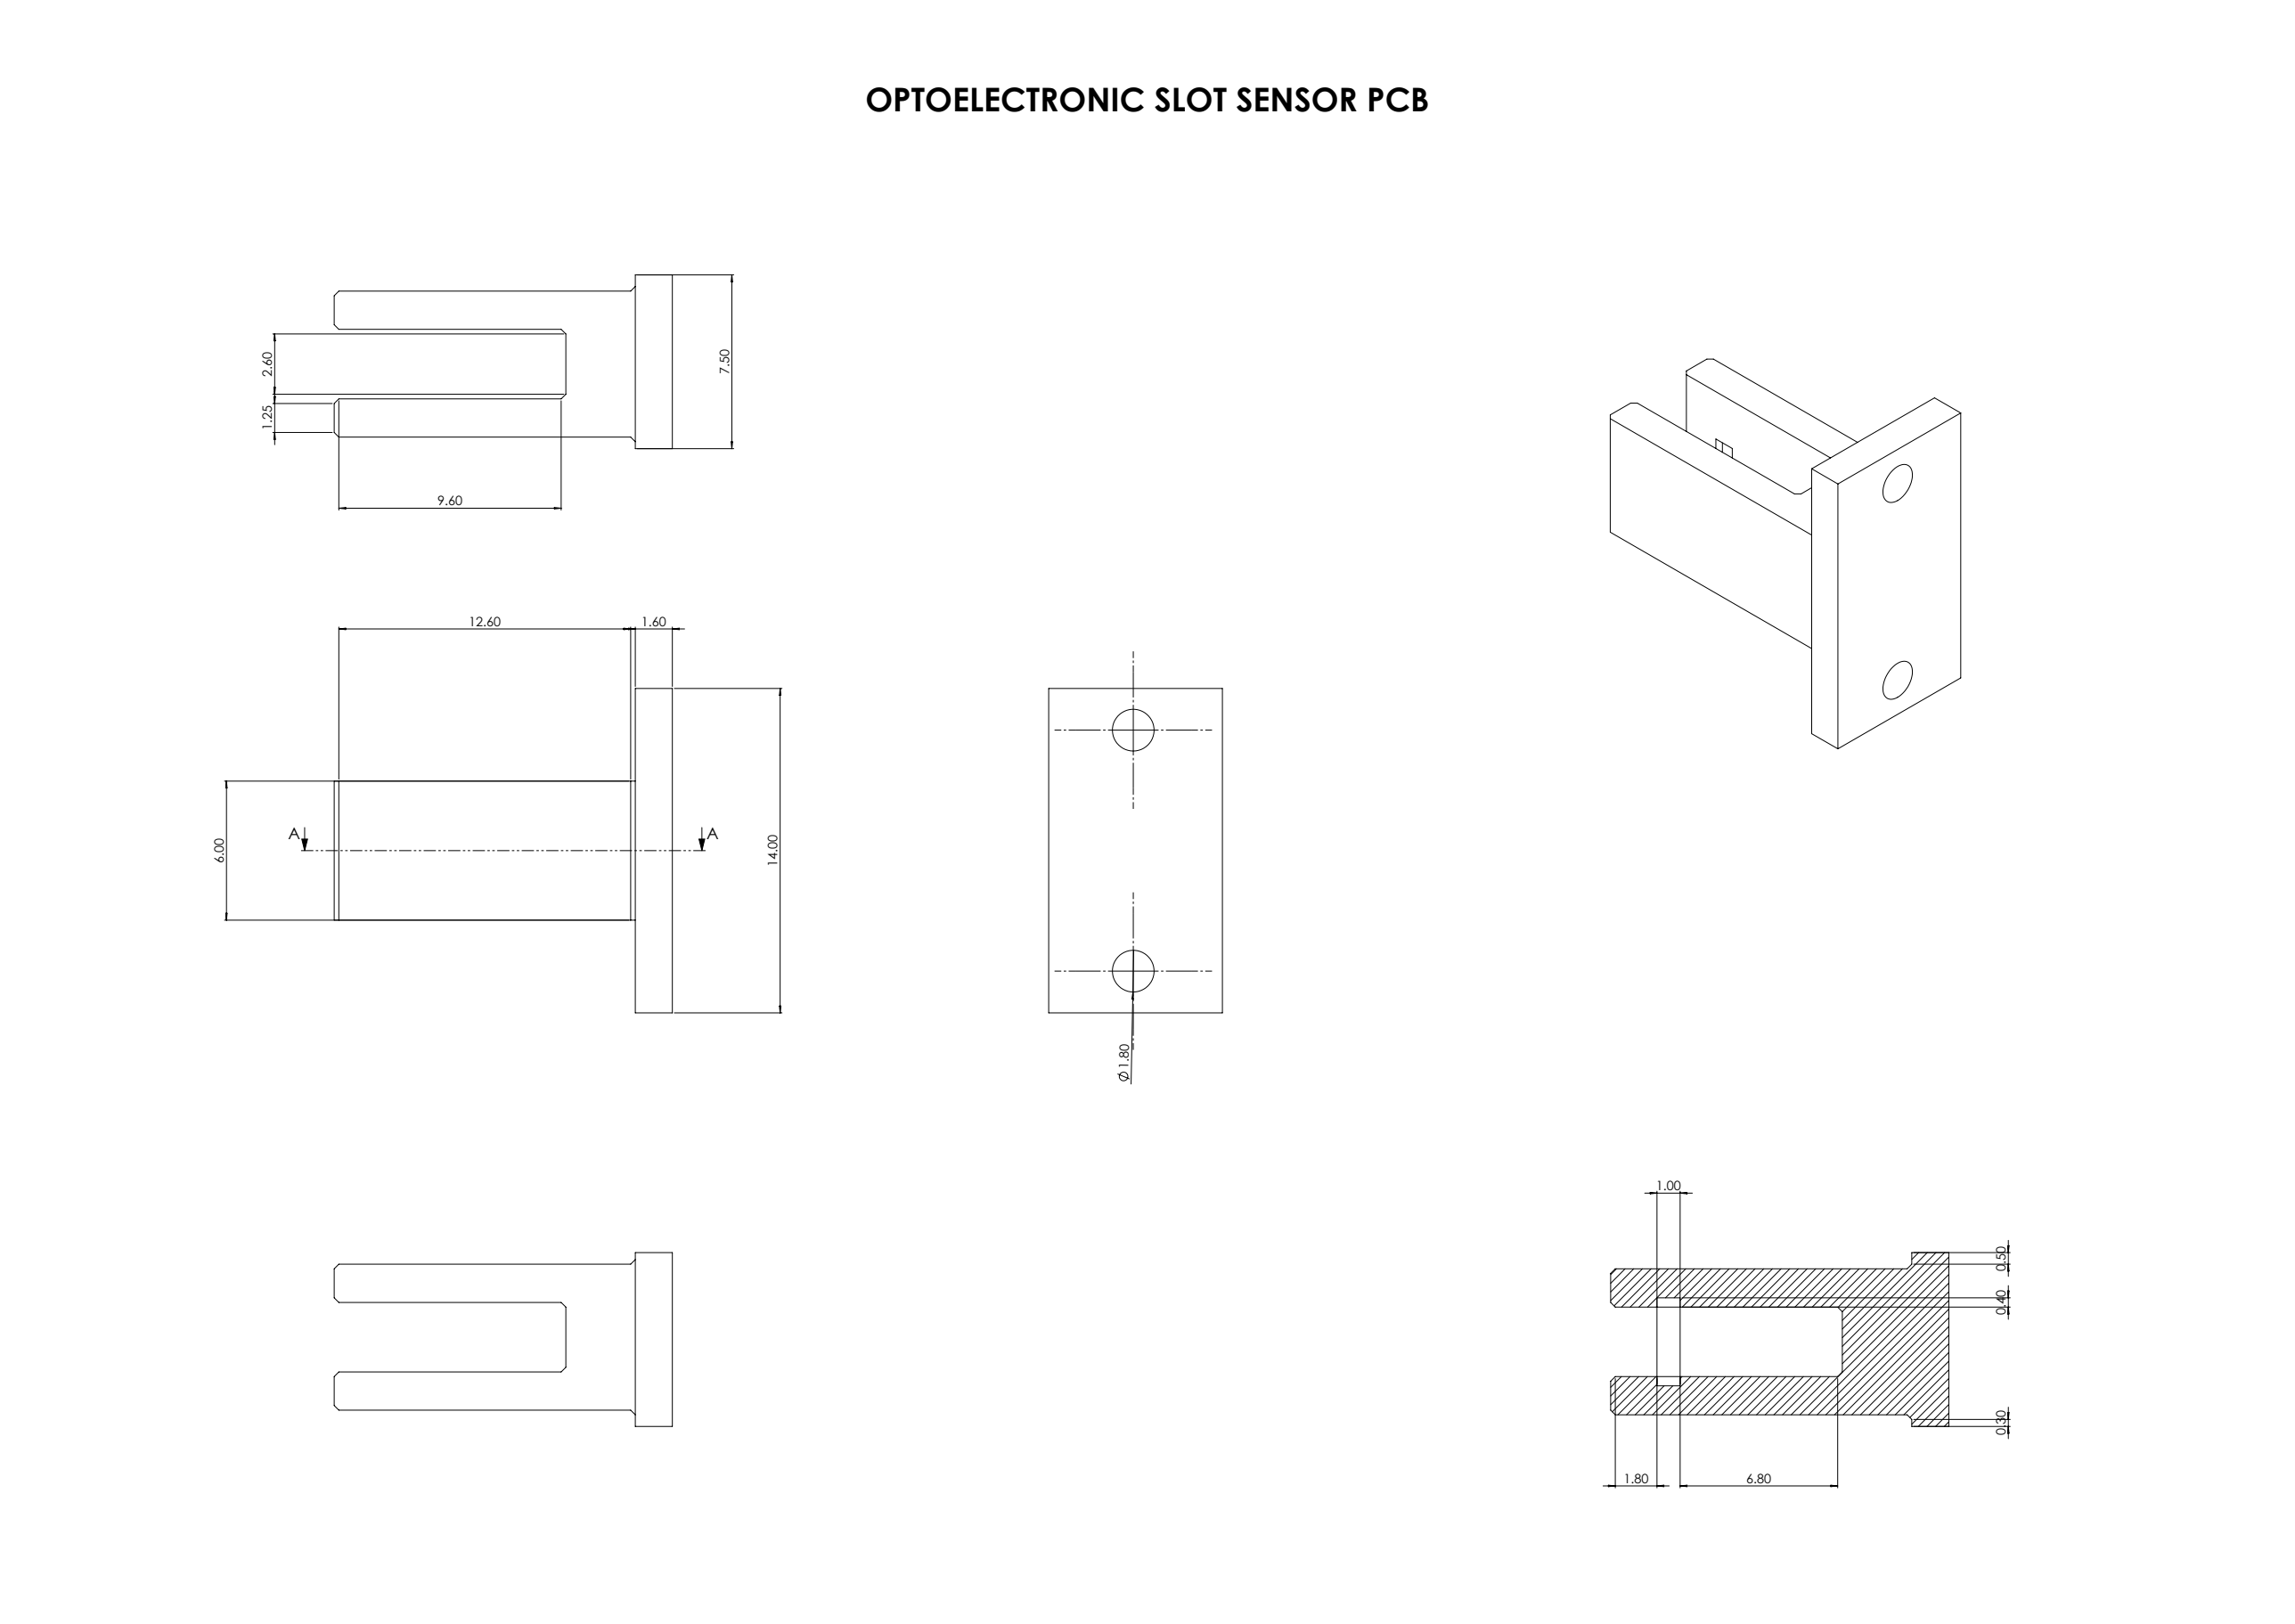
ISO-10303-21;
HEADER;
/* Generated by software containing ST-Developer
 * from STEP Tools, Inc. (www.steptools.com) 
 */

FILE_DESCRIPTION(
/* description */ (''),
/* implementation_level */ '2;1');

FILE_NAME(
/* name */ '11_Optoelectronic_Slot_Sensor_PCB.step',
/* time_stamp */ '2026-10-19T23:00:43-07:00',
/* author */ (''),
/* organization */ (''),
/* preprocessor_version */ 'ST-DEVELOPER v20.2',
/* originating_system */ 'Autodesk Translation Framework v15.15.0.0',
/* authorisation */ '');

FILE_SCHEMA (('AUTOMOTIVE_DESIGN { 1 0 10303 214 3 1 1 }'));
ENDSEC;

DATA;
#10=MECHANICAL_DESIGN_GEOMETRIC_PRESENTATION_REPRESENTATION('',(#1006),#55002);
#966=SHAPE_REPRESENTATION_RELATIONSHIP('SRR','None',#55114,#986);
#986=ADVANCED_BREP_SHAPE_REPRESENTATION('',(#1026),#54992);
#1006=STYLED_ITEM('',(#55379),#1026);
#1026=MANIFOLD_SOLID_BREP('Slot Sensor PCB',#24539);
#1232=FACE_BOUND('',#4568,.T.);
#1233=FACE_BOUND('',#4573,.T.);
#1234=FACE_BOUND('',#4577,.T.);
#1235=FACE_BOUND('',#4578,.T.);
#1236=FACE_BOUND('',#4579,.T.);
#1237=FACE_BOUND('',#4586,.T.);
#1238=FACE_BOUND('',#4587,.T.);
#1458=PLANE('',#26023);
#1459=PLANE('',#26024);
#1460=PLANE('',#26025);
#1461=PLANE('',#26026);
#1462=PLANE('',#26027);
#1463=PLANE('',#26028);
#1464=PLANE('',#26029);
#1465=PLANE('',#26030);
#1466=PLANE('',#26031);
#1467=PLANE('',#26032);
#1468=PLANE('',#26033);
#1469=PLANE('',#26034);
#1470=PLANE('',#26035);
#1471=PLANE('',#26036);
#1472=PLANE('',#26037);
#1473=PLANE('',#26040);
#1474=PLANE('',#26041);
#1475=PLANE('',#26046);
#1476=PLANE('',#26047);
#1477=PLANE('',#26048);
#1478=PLANE('',#26049);
#1479=PLANE('',#26050);
#1480=PLANE('',#26051);
#1481=PLANE('',#26052);
#1482=PLANE('',#26053);
#1483=PLANE('',#26054);
#1484=PLANE('',#26055);
#1485=PLANE('',#26056);
#1486=PLANE('',#26057);
#1487=PLANE('',#26058);
#1488=PLANE('',#26059);
#1489=PLANE('',#26060);
#1490=PLANE('',#26061);
#2178=CYLINDRICAL_SURFACE('',#26042,0.0900000000000001);
#2179=CYLINDRICAL_SURFACE('',#26044,0.09);
#3000=FACE_OUTER_BOUND('',#4560,.T.);
#3001=FACE_OUTER_BOUND('',#4561,.T.);
#3002=FACE_OUTER_BOUND('',#4562,.T.);
#3003=FACE_OUTER_BOUND('',#4563,.T.);
#3004=FACE_OUTER_BOUND('',#4564,.T.);
#3005=FACE_OUTER_BOUND('',#4565,.T.);
#3006=FACE_OUTER_BOUND('',#4566,.T.);
#3007=FACE_OUTER_BOUND('',#4567,.T.);
#3008=FACE_OUTER_BOUND('',#4569,.T.);
#3009=FACE_OUTER_BOUND('',#4570,.T.);
#3010=FACE_OUTER_BOUND('',#4571,.T.);
#3011=FACE_OUTER_BOUND('',#4572,.T.);
#3012=FACE_OUTER_BOUND('',#4574,.T.);
#3013=FACE_OUTER_BOUND('',#4575,.T.);
#3014=FACE_OUTER_BOUND('',#4576,.T.);
#3015=FACE_OUTER_BOUND('',#4580,.T.);
#3016=FACE_OUTER_BOUND('',#4581,.T.);
#3017=FACE_OUTER_BOUND('',#4582,.T.);
#3018=FACE_OUTER_BOUND('',#4583,.T.);
#3019=FACE_OUTER_BOUND('',#4584,.T.);
#3020=FACE_OUTER_BOUND('',#4585,.T.);
#3021=FACE_OUTER_BOUND('',#4588,.T.);
#3022=FACE_OUTER_BOUND('',#4589,.T.);
#3023=FACE_OUTER_BOUND('',#4590,.T.);
#3024=FACE_OUTER_BOUND('',#4591,.T.);
#3025=FACE_OUTER_BOUND('',#4592,.T.);
#3026=FACE_OUTER_BOUND('',#4593,.T.);
#3027=FACE_OUTER_BOUND('',#4594,.T.);
#3028=FACE_OUTER_BOUND('',#4595,.T.);
#3029=FACE_OUTER_BOUND('',#4596,.T.);
#3030=FACE_OUTER_BOUND('',#4597,.T.);
#3031=FACE_OUTER_BOUND('',#4598,.T.);
#3032=FACE_OUTER_BOUND('',#4599,.T.);
#3033=FACE_OUTER_BOUND('',#4600,.T.);
#3034=FACE_OUTER_BOUND('',#4601,.T.);
#4560=EDGE_LOOP('',(#18604,#18605,#18606,#18607));
#4561=EDGE_LOOP('',(#18608,#18609,#18610,#18611));
#4562=EDGE_LOOP('',(#18612,#18613,#18614,#18615,#18616,#18617,#18618,#18619,
#18620,#18621,#18622,#18623,#18624,#18625,#18626,#18627));
#4563=EDGE_LOOP('',(#18628,#18629,#18630,#18631));
#4564=EDGE_LOOP('',(#18632,#18633,#18634,#18635));
#4565=EDGE_LOOP('',(#18636,#18637,#18638,#18639,#18640,#18641,#18642,#18643,
#18644,#18645,#18646,#18647,#18648,#18649,#18650,#18651));
#4566=EDGE_LOOP('',(#18652,#18653,#18654,#18655));
#4567=EDGE_LOOP('',(#18656,#18657,#18658,#18659));
#4568=EDGE_LOOP('',(#18660,#18661,#18662,#18663));
#4569=EDGE_LOOP('',(#18664,#18665,#18666,#18667));
#4570=EDGE_LOOP('',(#18668,#18669,#18670,#18671));
#4571=EDGE_LOOP('',(#18672,#18673,#18674,#18675));
#4572=EDGE_LOOP('',(#18676,#18677,#18678,#18679));
#4573=EDGE_LOOP('',(#18680,#18681,#18682,#18683));
#4574=EDGE_LOOP('',(#18684,#18685,#18686,#18687));
#4575=EDGE_LOOP('',(#18688,#18689,#18690,#18691));
#4576=EDGE_LOOP('',(#18692,#18693,#18694,#18695));
#4577=EDGE_LOOP('',(#18696));
#4578=EDGE_LOOP('',(#18697));
#4579=EDGE_LOOP('',(#18698,#18699,#18700,#18701));
#4580=EDGE_LOOP('',(#18702,#18703,#18704,#18705));
#4581=EDGE_LOOP('',(#18706,#18707,#18708,#18709));
#4582=EDGE_LOOP('',(#18710,#18711,#18712,#18713));
#4583=EDGE_LOOP('',(#18714,#18715,#18716,#18717));
#4584=EDGE_LOOP('',(#18718,#18719,#18720,#18721));
#4585=EDGE_LOOP('',(#18722,#18723,#18724,#18725));
#4586=EDGE_LOOP('',(#18726));
#4587=EDGE_LOOP('',(#18727));
#4588=EDGE_LOOP('',(#18728,#18729,#18730,#18731));
#4589=EDGE_LOOP('',(#18732,#18733,#18734,#18735));
#4590=EDGE_LOOP('',(#18736,#18737,#18738,#18739));
#4591=EDGE_LOOP('',(#18740,#18741,#18742,#18743));
#4592=EDGE_LOOP('',(#18744,#18745,#18746,#18747));
#4593=EDGE_LOOP('',(#18748,#18749,#18750,#18751));
#4594=EDGE_LOOP('',(#18752,#18753,#18754,#18755));
#4595=EDGE_LOOP('',(#18756,#18757,#18758,#18759));
#4596=EDGE_LOOP('',(#18760,#18761,#18762,#18763));
#4597=EDGE_LOOP('',(#18764,#18765,#18766,#18767));
#4598=EDGE_LOOP('',(#18768,#18769,#18770,#18771));
#4599=EDGE_LOOP('',(#18772,#18773,#18774,#18775));
#4600=EDGE_LOOP('',(#18776,#18777,#18778,#18779));
#4601=EDGE_LOOP('',(#18780,#18781,#18782,#18783));
#6062=LINE('',#37264,#7883);
#6063=LINE('',#37266,#7884);
#6064=LINE('',#37268,#7885);
#6065=LINE('',#37269,#7886);
#6066=LINE('',#37272,#7887);
#6067=LINE('',#37274,#7888);
#6068=LINE('',#37275,#7889);
#6069=LINE('',#37278,#7890);
#6070=LINE('',#37280,#7891);
#6071=LINE('',#37282,#7892);
#6072=LINE('',#37284,#7893);
#6073=LINE('',#37286,#7894);
#6074=LINE('',#37288,#7895);
#6075=LINE('',#37290,#7896);
#6076=LINE('',#37292,#7897);
#6077=LINE('',#37294,#7898);
#6078=LINE('',#37296,#7899);
#6079=LINE('',#37298,#7900);
#6080=LINE('',#37300,#7901);
#6081=LINE('',#37302,#7902);
#6082=LINE('',#37303,#7903);
#6083=LINE('',#37306,#7904);
#6084=LINE('',#37308,#7905);
#6085=LINE('',#37309,#7906);
#6086=LINE('',#37312,#7907);
#6087=LINE('',#37313,#7908);
#6088=LINE('',#37316,#7909);
#6089=LINE('',#37318,#7910);
#6090=LINE('',#37320,#7911);
#6091=LINE('',#37322,#7912);
#6092=LINE('',#37324,#7913);
#6093=LINE('',#37326,#7914);
#6094=LINE('',#37327,#7915);
#6095=LINE('',#37329,#7916);
#6096=LINE('',#37331,#7917);
#6097=LINE('',#37333,#7918);
#6098=LINE('',#37335,#7919);
#6099=LINE('',#37336,#7920);
#6100=LINE('',#37338,#7921);
#6101=LINE('',#37340,#7922);
#6102=LINE('',#37343,#7923);
#6103=LINE('',#37345,#7924);
#6104=LINE('',#37347,#7925);
#6105=LINE('',#37348,#7926);
#6106=LINE('',#37350,#7927);
#6107=LINE('',#37352,#7928);
#6108=LINE('',#37354,#7929);
#6109=LINE('',#37356,#7930);
#6110=LINE('',#37359,#7931);
#6111=LINE('',#37361,#7932);
#6112=LINE('',#37363,#7933);
#6113=LINE('',#37364,#7934);
#6114=LINE('',#37367,#7935);
#6115=LINE('',#37368,#7936);
#6116=LINE('',#37372,#7937);
#6117=LINE('',#37374,#7938);
#6118=LINE('',#37376,#7939);
#6119=LINE('',#37377,#7940);
#6120=LINE('',#37382,#7941);
#6121=LINE('',#37384,#7942);
#6122=LINE('',#37389,#7943);
#6123=LINE('',#37393,#7944);
#6124=LINE('',#37396,#7945);
#6125=LINE('',#37398,#7946);
#6126=LINE('',#37399,#7947);
#6127=LINE('',#37402,#7948);
#6128=LINE('',#37404,#7949);
#6129=LINE('',#37405,#7950);
#6130=LINE('',#37407,#7951);
#6131=LINE('',#37408,#7952);
#6132=LINE('',#37414,#7953);
#6133=LINE('',#37415,#7954);
#6134=LINE('',#37416,#7955);
#6135=LINE('',#37419,#7956);
#6136=LINE('',#37420,#7957);
#6137=LINE('',#37423,#7958);
#6138=LINE('',#37424,#7959);
#6139=LINE('',#37426,#7960);
#6140=LINE('',#37430,#7961);
#6141=LINE('',#37432,#7962);
#6142=LINE('',#37433,#7963);
#6143=LINE('',#37436,#7964);
#6144=LINE('',#37437,#7965);
#6145=LINE('',#37440,#7966);
#6146=LINE('',#37441,#7967);
#6147=LINE('',#37443,#7968);
#7883=VECTOR('',#30386,1.);
#7884=VECTOR('',#30387,1.);
#7885=VECTOR('',#30388,1.);
#7886=VECTOR('',#30389,1.);
#7887=VECTOR('',#30392,1.);
#7888=VECTOR('',#30393,1.);
#7889=VECTOR('',#30394,1.);
#7890=VECTOR('',#30397,1.);
#7891=VECTOR('',#30398,1.);
#7892=VECTOR('',#30399,1.);
#7893=VECTOR('',#30400,1.);
#7894=VECTOR('',#30401,1.);
#7895=VECTOR('',#30402,1.);
#7896=VECTOR('',#30403,1.);
#7897=VECTOR('',#30404,1.);
#7898=VECTOR('',#30405,1.);
#7899=VECTOR('',#30406,1.);
#7900=VECTOR('',#30407,1.);
#7901=VECTOR('',#30408,1.);
#7902=VECTOR('',#30409,1.);
#7903=VECTOR('',#30410,1.);
#7904=VECTOR('',#30413,1.);
#7905=VECTOR('',#30414,1.);
#7906=VECTOR('',#30415,1.);
#7907=VECTOR('',#30418,1.);
#7908=VECTOR('',#30419,1.);
#7909=VECTOR('',#30422,1.);
#7910=VECTOR('',#30423,1.);
#7911=VECTOR('',#30424,1.);
#7912=VECTOR('',#30425,1.);
#7913=VECTOR('',#30426,1.);
#7914=VECTOR('',#30427,1.);
#7915=VECTOR('',#30428,1.);
#7916=VECTOR('',#30429,1.);
#7917=VECTOR('',#30430,1.);
#7918=VECTOR('',#30431,1.);
#7919=VECTOR('',#30432,1.);
#7920=VECTOR('',#30433,1.);
#7921=VECTOR('',#30436,1.);
#7922=VECTOR('',#30439,1.);
#7923=VECTOR('',#30440,1.);
#7924=VECTOR('',#30441,1.);
#7925=VECTOR('',#30442,1.);
#7926=VECTOR('',#30443,1.);
#7927=VECTOR('',#30446,1.);
#7928=VECTOR('',#30449,1.);
#7929=VECTOR('',#30452,1.);
#7930=VECTOR('',#30455,1.);
#7931=VECTOR('',#30456,1.);
#7932=VECTOR('',#30457,1.);
#7933=VECTOR('',#30458,1.);
#7934=VECTOR('',#30459,1.);
#7935=VECTOR('',#30464,1.);
#7936=VECTOR('',#30465,1.);
#7937=VECTOR('',#30468,1.);
#7938=VECTOR('',#30469,1.);
#7939=VECTOR('',#30470,1.);
#7940=VECTOR('',#30471,1.);
#7941=VECTOR('',#30476,1.);
#7942=VECTOR('',#30479,1.);
#7943=VECTOR('',#30486,0.0900000000000001);
#7944=VECTOR('',#30491,0.09);
#7945=VECTOR('',#30494,1.);
#7946=VECTOR('',#30495,1.);
#7947=VECTOR('',#30496,1.);
#7948=VECTOR('',#30499,1.);
#7949=VECTOR('',#30500,1.);
#7950=VECTOR('',#30501,1.);
#7951=VECTOR('',#30504,1.);
#7952=VECTOR('',#30505,1.);
#7953=VECTOR('',#30512,1.);
#7954=VECTOR('',#30513,1.);
#7955=VECTOR('',#30514,1.);
#7956=VECTOR('',#30517,1.);
#7957=VECTOR('',#30518,1.);
#7958=VECTOR('',#30521,1.);
#7959=VECTOR('',#30522,1.);
#7960=VECTOR('',#30525,1.);
#7961=VECTOR('',#30530,1.);
#7962=VECTOR('',#30531,1.);
#7963=VECTOR('',#30532,1.);
#7964=VECTOR('',#30535,1.);
#7965=VECTOR('',#30536,1.);
#7966=VECTOR('',#30539,1.);
#7967=VECTOR('',#30540,1.);
#7968=VECTOR('',#30543,1.);
#9678=CIRCLE('',#26038,0.09);
#9679=CIRCLE('',#26039,0.0900000000000001);
#9680=CIRCLE('',#26043,0.0900000000000001);
#9681=CIRCLE('',#26045,0.09);
#10905=VERTEX_POINT('',#37262);
#10906=VERTEX_POINT('',#37263);
#10907=VERTEX_POINT('',#37265);
#10908=VERTEX_POINT('',#37267);
#10909=VERTEX_POINT('',#37271);
#10910=VERTEX_POINT('',#37273);
#10911=VERTEX_POINT('',#37277);
#10912=VERTEX_POINT('',#37279);
#10913=VERTEX_POINT('',#37281);
#10914=VERTEX_POINT('',#37283);
#10915=VERTEX_POINT('',#37285);
#10916=VERTEX_POINT('',#37287);
#10917=VERTEX_POINT('',#37289);
#10918=VERTEX_POINT('',#37291);
#10919=VERTEX_POINT('',#37293);
#10920=VERTEX_POINT('',#37295);
#10921=VERTEX_POINT('',#37297);
#10922=VERTEX_POINT('',#37299);
#10923=VERTEX_POINT('',#37301);
#10924=VERTEX_POINT('',#37305);
#10925=VERTEX_POINT('',#37307);
#10926=VERTEX_POINT('',#37311);
#10927=VERTEX_POINT('',#37315);
#10928=VERTEX_POINT('',#37317);
#10929=VERTEX_POINT('',#37319);
#10930=VERTEX_POINT('',#37321);
#10931=VERTEX_POINT('',#37323);
#10932=VERTEX_POINT('',#37325);
#10933=VERTEX_POINT('',#37328);
#10934=VERTEX_POINT('',#37330);
#10935=VERTEX_POINT('',#37332);
#10936=VERTEX_POINT('',#37334);
#10937=VERTEX_POINT('',#37341);
#10938=VERTEX_POINT('',#37342);
#10939=VERTEX_POINT('',#37344);
#10940=VERTEX_POINT('',#37346);
#10941=VERTEX_POINT('',#37357);
#10942=VERTEX_POINT('',#37358);
#10943=VERTEX_POINT('',#37360);
#10944=VERTEX_POINT('',#37362);
#10945=VERTEX_POINT('',#37370);
#10946=VERTEX_POINT('',#37371);
#10947=VERTEX_POINT('',#37373);
#10948=VERTEX_POINT('',#37375);
#10949=VERTEX_POINT('',#37378);
#10950=VERTEX_POINT('',#37380);
#10951=VERTEX_POINT('',#37387);
#10952=VERTEX_POINT('',#37391);
#10953=VERTEX_POINT('',#37395);
#10954=VERTEX_POINT('',#37397);
#10955=VERTEX_POINT('',#37401);
#10956=VERTEX_POINT('',#37403);
#10957=VERTEX_POINT('',#37412);
#10958=VERTEX_POINT('',#37413);
#10959=VERTEX_POINT('',#37418);
#10960=VERTEX_POINT('',#37422);
#10961=VERTEX_POINT('',#37429);
#10962=VERTEX_POINT('',#37431);
#10963=VERTEX_POINT('',#37435);
#10964=VERTEX_POINT('',#37439);
#13710=EDGE_CURVE('',#10905,#10906,#6062,.T.);
#13711=EDGE_CURVE('',#10906,#10907,#6063,.T.);
#13712=EDGE_CURVE('',#10907,#10908,#6064,.T.);
#13713=EDGE_CURVE('',#10908,#10905,#6065,.T.);
#13714=EDGE_CURVE('',#10906,#10909,#6066,.T.);
#13715=EDGE_CURVE('',#10910,#10909,#6067,.T.);
#13716=EDGE_CURVE('',#10907,#10910,#6068,.T.);
#13717=EDGE_CURVE('',#10905,#10911,#6069,.T.);
#13718=EDGE_CURVE('',#10912,#10911,#6070,.T.);
#13719=EDGE_CURVE('',#10912,#10913,#6071,.T.);
#13720=EDGE_CURVE('',#10914,#10913,#6072,.T.);
#13721=EDGE_CURVE('',#10915,#10914,#6073,.T.);
#13722=EDGE_CURVE('',#10916,#10915,#6074,.T.);
#13723=EDGE_CURVE('',#10917,#10916,#6075,.T.);
#13724=EDGE_CURVE('',#10918,#10917,#6076,.T.);
#13725=EDGE_CURVE('',#10918,#10919,#6077,.T.);
#13726=EDGE_CURVE('',#10920,#10919,#6078,.T.);
#13727=EDGE_CURVE('',#10920,#10921,#6079,.T.);
#13728=EDGE_CURVE('',#10922,#10921,#6080,.T.);
#13729=EDGE_CURVE('',#10922,#10923,#6081,.T.);
#13730=EDGE_CURVE('',#10909,#10923,#6082,.T.);
#13731=EDGE_CURVE('',#10915,#10924,#6083,.T.);
#13732=EDGE_CURVE('',#10924,#10925,#6084,.T.);
#13733=EDGE_CURVE('',#10925,#10916,#6085,.T.);
#13734=EDGE_CURVE('',#10926,#10925,#6086,.T.);
#13735=EDGE_CURVE('',#10917,#10926,#6087,.T.);
#13736=EDGE_CURVE('',#10927,#10910,#6088,.T.);
#13737=EDGE_CURVE('',#10927,#10928,#6089,.T.);
#13738=EDGE_CURVE('',#10929,#10928,#6090,.T.);
#13739=EDGE_CURVE('',#10929,#10930,#6091,.T.);
#13740=EDGE_CURVE('',#10931,#10930,#6092,.T.);
#13741=EDGE_CURVE('',#10931,#10932,#6093,.T.);
#13742=EDGE_CURVE('',#10926,#10932,#6094,.T.);
#13743=EDGE_CURVE('',#10933,#10924,#6095,.T.);
#13744=EDGE_CURVE('',#10934,#10933,#6096,.T.);
#13745=EDGE_CURVE('',#10935,#10934,#6097,.T.);
#13746=EDGE_CURVE('',#10936,#10935,#6098,.T.);
#13747=EDGE_CURVE('',#10936,#10908,#6099,.T.);
#13748=EDGE_CURVE('',#10923,#10927,#6100,.T.);
#13749=EDGE_CURVE('',#10928,#10922,#6101,.T.);
#13750=EDGE_CURVE('',#10937,#10938,#6102,.T.);
#13751=EDGE_CURVE('',#10938,#10939,#6103,.T.);
#13752=EDGE_CURVE('',#10939,#10940,#6104,.T.);
#13753=EDGE_CURVE('',#10940,#10937,#6105,.T.);
#13754=EDGE_CURVE('',#10921,#10929,#6106,.T.);
#13755=EDGE_CURVE('',#10930,#10920,#6107,.T.);
#13756=EDGE_CURVE('',#10932,#10918,#6108,.T.);
#13757=EDGE_CURVE('',#10919,#10931,#6109,.T.);
#13758=EDGE_CURVE('',#10941,#10942,#6110,.T.);
#13759=EDGE_CURVE('',#10942,#10943,#6111,.T.);
#13760=EDGE_CURVE('',#10943,#10944,#6112,.T.);
#13761=EDGE_CURVE('',#10944,#10941,#6113,.T.);
#13762=EDGE_CURVE('',#10913,#10934,#6114,.T.);
#13763=EDGE_CURVE('',#10933,#10914,#6115,.T.);
#13764=EDGE_CURVE('',#10945,#10946,#6116,.T.);
#13765=EDGE_CURVE('',#10946,#10947,#6117,.T.);
#13766=EDGE_CURVE('',#10948,#10947,#6118,.T.);
#13767=EDGE_CURVE('',#10945,#10948,#6119,.T.);
#13768=EDGE_CURVE('',#10949,#10949,#9678,.T.);
#13769=EDGE_CURVE('',#10950,#10950,#9679,.T.);
#13770=EDGE_CURVE('',#10935,#10912,#6120,.T.);
#13771=EDGE_CURVE('',#10911,#10936,#6121,.T.);
#13772=EDGE_CURVE('',#10951,#10951,#9680,.T.);
#13773=EDGE_CURVE('',#10951,#10950,#6122,.T.);
#13774=EDGE_CURVE('',#10952,#10952,#9681,.T.);
#13775=EDGE_CURVE('',#10952,#10949,#6123,.T.);
#13776=EDGE_CURVE('',#10953,#10945,#6124,.T.);
#13777=EDGE_CURVE('',#10954,#10948,#6125,.T.);
#13778=EDGE_CURVE('',#10953,#10954,#6126,.T.);
#13779=EDGE_CURVE('',#10955,#10953,#6127,.T.);
#13780=EDGE_CURVE('',#10956,#10954,#6128,.T.);
#13781=EDGE_CURVE('',#10955,#10956,#6129,.T.);
#13782=EDGE_CURVE('',#10946,#10955,#6130,.T.);
#13783=EDGE_CURVE('',#10947,#10956,#6131,.T.);
#13784=EDGE_CURVE('',#10957,#10958,#6132,.T.);
#13785=EDGE_CURVE('',#10957,#10938,#6133,.T.);
#13786=EDGE_CURVE('',#10958,#10937,#6134,.T.);
#13787=EDGE_CURVE('',#10959,#10957,#6135,.T.);
#13788=EDGE_CURVE('',#10959,#10939,#6136,.T.);
#13789=EDGE_CURVE('',#10960,#10959,#6137,.T.);
#13790=EDGE_CURVE('',#10960,#10940,#6138,.T.);
#13791=EDGE_CURVE('',#10958,#10960,#6139,.T.);
#13792=EDGE_CURVE('',#10941,#10961,#6140,.T.);
#13793=EDGE_CURVE('',#10961,#10962,#6141,.T.);
#13794=EDGE_CURVE('',#10942,#10962,#6142,.T.);
#13795=EDGE_CURVE('',#10944,#10963,#6143,.T.);
#13796=EDGE_CURVE('',#10963,#10961,#6144,.T.);
#13797=EDGE_CURVE('',#10943,#10964,#6145,.T.);
#13798=EDGE_CURVE('',#10964,#10963,#6146,.T.);
#13799=EDGE_CURVE('',#10962,#10964,#6147,.T.);
#18604=ORIENTED_EDGE('',*,*,#13710,.T.);
#18605=ORIENTED_EDGE('',*,*,#13711,.T.);
#18606=ORIENTED_EDGE('',*,*,#13712,.T.);
#18607=ORIENTED_EDGE('',*,*,#13713,.T.);
#18608=ORIENTED_EDGE('',*,*,#13711,.F.);
#18609=ORIENTED_EDGE('',*,*,#13714,.T.);
#18610=ORIENTED_EDGE('',*,*,#13715,.F.);
#18611=ORIENTED_EDGE('',*,*,#13716,.F.);
#18612=ORIENTED_EDGE('',*,*,#13710,.F.);
#18613=ORIENTED_EDGE('',*,*,#13717,.T.);
#18614=ORIENTED_EDGE('',*,*,#13718,.F.);
#18615=ORIENTED_EDGE('',*,*,#13719,.T.);
#18616=ORIENTED_EDGE('',*,*,#13720,.F.);
#18617=ORIENTED_EDGE('',*,*,#13721,.F.);
#18618=ORIENTED_EDGE('',*,*,#13722,.F.);
#18619=ORIENTED_EDGE('',*,*,#13723,.F.);
#18620=ORIENTED_EDGE('',*,*,#13724,.F.);
#18621=ORIENTED_EDGE('',*,*,#13725,.T.);
#18622=ORIENTED_EDGE('',*,*,#13726,.F.);
#18623=ORIENTED_EDGE('',*,*,#13727,.T.);
#18624=ORIENTED_EDGE('',*,*,#13728,.F.);
#18625=ORIENTED_EDGE('',*,*,#13729,.T.);
#18626=ORIENTED_EDGE('',*,*,#13730,.F.);
#18627=ORIENTED_EDGE('',*,*,#13714,.F.);
#18628=ORIENTED_EDGE('',*,*,#13722,.T.);
#18629=ORIENTED_EDGE('',*,*,#13731,.T.);
#18630=ORIENTED_EDGE('',*,*,#13732,.T.);
#18631=ORIENTED_EDGE('',*,*,#13733,.T.);
#18632=ORIENTED_EDGE('',*,*,#13733,.F.);
#18633=ORIENTED_EDGE('',*,*,#13734,.F.);
#18634=ORIENTED_EDGE('',*,*,#13735,.F.);
#18635=ORIENTED_EDGE('',*,*,#13723,.T.);
#18636=ORIENTED_EDGE('',*,*,#13712,.F.);
#18637=ORIENTED_EDGE('',*,*,#13716,.T.);
#18638=ORIENTED_EDGE('',*,*,#13736,.F.);
#18639=ORIENTED_EDGE('',*,*,#13737,.T.);
#18640=ORIENTED_EDGE('',*,*,#13738,.F.);
#18641=ORIENTED_EDGE('',*,*,#13739,.T.);
#18642=ORIENTED_EDGE('',*,*,#13740,.F.);
#18643=ORIENTED_EDGE('',*,*,#13741,.T.);
#18644=ORIENTED_EDGE('',*,*,#13742,.F.);
#18645=ORIENTED_EDGE('',*,*,#13734,.T.);
#18646=ORIENTED_EDGE('',*,*,#13732,.F.);
#18647=ORIENTED_EDGE('',*,*,#13743,.F.);
#18648=ORIENTED_EDGE('',*,*,#13744,.F.);
#18649=ORIENTED_EDGE('',*,*,#13745,.F.);
#18650=ORIENTED_EDGE('',*,*,#13746,.F.);
#18651=ORIENTED_EDGE('',*,*,#13747,.T.);
#18652=ORIENTED_EDGE('',*,*,#13736,.T.);
#18653=ORIENTED_EDGE('',*,*,#13715,.T.);
#18654=ORIENTED_EDGE('',*,*,#13730,.T.);
#18655=ORIENTED_EDGE('',*,*,#13748,.T.);
#18656=ORIENTED_EDGE('',*,*,#13748,.F.);
#18657=ORIENTED_EDGE('',*,*,#13729,.F.);
#18658=ORIENTED_EDGE('',*,*,#13749,.F.);
#18659=ORIENTED_EDGE('',*,*,#13737,.F.);
#18660=ORIENTED_EDGE('',*,*,#13750,.T.);
#18661=ORIENTED_EDGE('',*,*,#13751,.T.);
#18662=ORIENTED_EDGE('',*,*,#13752,.T.);
#18663=ORIENTED_EDGE('',*,*,#13753,.T.);
#18664=ORIENTED_EDGE('',*,*,#13728,.T.);
#18665=ORIENTED_EDGE('',*,*,#13754,.T.);
#18666=ORIENTED_EDGE('',*,*,#13738,.T.);
#18667=ORIENTED_EDGE('',*,*,#13749,.T.);
#18668=ORIENTED_EDGE('',*,*,#13754,.F.);
#18669=ORIENTED_EDGE('',*,*,#13727,.F.);
#18670=ORIENTED_EDGE('',*,*,#13755,.F.);
#18671=ORIENTED_EDGE('',*,*,#13739,.F.);
#18672=ORIENTED_EDGE('',*,*,#13724,.T.);
#18673=ORIENTED_EDGE('',*,*,#13735,.T.);
#18674=ORIENTED_EDGE('',*,*,#13742,.T.);
#18675=ORIENTED_EDGE('',*,*,#13756,.T.);
#18676=ORIENTED_EDGE('',*,*,#13756,.F.);
#18677=ORIENTED_EDGE('',*,*,#13741,.F.);
#18678=ORIENTED_EDGE('',*,*,#13757,.F.);
#18679=ORIENTED_EDGE('',*,*,#13725,.F.);
#18680=ORIENTED_EDGE('',*,*,#13758,.T.);
#18681=ORIENTED_EDGE('',*,*,#13759,.T.);
#18682=ORIENTED_EDGE('',*,*,#13760,.T.);
#18683=ORIENTED_EDGE('',*,*,#13761,.T.);
#18684=ORIENTED_EDGE('',*,*,#13726,.T.);
#18685=ORIENTED_EDGE('',*,*,#13757,.T.);
#18686=ORIENTED_EDGE('',*,*,#13740,.T.);
#18687=ORIENTED_EDGE('',*,*,#13755,.T.);
#18688=ORIENTED_EDGE('',*,*,#13720,.T.);
#18689=ORIENTED_EDGE('',*,*,#13762,.T.);
#18690=ORIENTED_EDGE('',*,*,#13744,.T.);
#18691=ORIENTED_EDGE('',*,*,#13763,.T.);
#18692=ORIENTED_EDGE('',*,*,#13764,.T.);
#18693=ORIENTED_EDGE('',*,*,#13765,.T.);
#18694=ORIENTED_EDGE('',*,*,#13766,.F.);
#18695=ORIENTED_EDGE('',*,*,#13767,.F.);
#18696=ORIENTED_EDGE('',*,*,#13768,.T.);
#18697=ORIENTED_EDGE('',*,*,#13769,.T.);
#18698=ORIENTED_EDGE('',*,*,#13745,.T.);
#18699=ORIENTED_EDGE('',*,*,#13762,.F.);
#18700=ORIENTED_EDGE('',*,*,#13719,.F.);
#18701=ORIENTED_EDGE('',*,*,#13770,.F.);
#18702=ORIENTED_EDGE('',*,*,#13718,.T.);
#18703=ORIENTED_EDGE('',*,*,#13771,.T.);
#18704=ORIENTED_EDGE('',*,*,#13746,.T.);
#18705=ORIENTED_EDGE('',*,*,#13770,.T.);
#18706=ORIENTED_EDGE('',*,*,#13713,.F.);
#18707=ORIENTED_EDGE('',*,*,#13747,.F.);
#18708=ORIENTED_EDGE('',*,*,#13771,.F.);
#18709=ORIENTED_EDGE('',*,*,#13717,.F.);
#18710=ORIENTED_EDGE('',*,*,#13772,.F.);
#18711=ORIENTED_EDGE('',*,*,#13773,.T.);
#18712=ORIENTED_EDGE('',*,*,#13769,.F.);
#18713=ORIENTED_EDGE('',*,*,#13773,.F.);
#18714=ORIENTED_EDGE('',*,*,#13774,.F.);
#18715=ORIENTED_EDGE('',*,*,#13775,.T.);
#18716=ORIENTED_EDGE('',*,*,#13768,.F.);
#18717=ORIENTED_EDGE('',*,*,#13775,.F.);
#18718=ORIENTED_EDGE('',*,*,#13776,.T.);
#18719=ORIENTED_EDGE('',*,*,#13767,.T.);
#18720=ORIENTED_EDGE('',*,*,#13777,.F.);
#18721=ORIENTED_EDGE('',*,*,#13778,.F.);
#18722=ORIENTED_EDGE('',*,*,#13779,.T.);
#18723=ORIENTED_EDGE('',*,*,#13778,.T.);
#18724=ORIENTED_EDGE('',*,*,#13780,.F.);
#18725=ORIENTED_EDGE('',*,*,#13781,.F.);
#18726=ORIENTED_EDGE('',*,*,#13772,.T.);
#18727=ORIENTED_EDGE('',*,*,#13774,.T.);
#18728=ORIENTED_EDGE('',*,*,#13782,.T.);
#18729=ORIENTED_EDGE('',*,*,#13781,.T.);
#18730=ORIENTED_EDGE('',*,*,#13783,.F.);
#18731=ORIENTED_EDGE('',*,*,#13765,.F.);
#18732=ORIENTED_EDGE('',*,*,#13766,.T.);
#18733=ORIENTED_EDGE('',*,*,#13783,.T.);
#18734=ORIENTED_EDGE('',*,*,#13780,.T.);
#18735=ORIENTED_EDGE('',*,*,#13777,.T.);
#18736=ORIENTED_EDGE('',*,*,#13764,.F.);
#18737=ORIENTED_EDGE('',*,*,#13776,.F.);
#18738=ORIENTED_EDGE('',*,*,#13779,.F.);
#18739=ORIENTED_EDGE('',*,*,#13782,.F.);
#18740=ORIENTED_EDGE('',*,*,#13784,.F.);
#18741=ORIENTED_EDGE('',*,*,#13785,.T.);
#18742=ORIENTED_EDGE('',*,*,#13750,.F.);
#18743=ORIENTED_EDGE('',*,*,#13786,.F.);
#18744=ORIENTED_EDGE('',*,*,#13787,.F.);
#18745=ORIENTED_EDGE('',*,*,#13788,.T.);
#18746=ORIENTED_EDGE('',*,*,#13751,.F.);
#18747=ORIENTED_EDGE('',*,*,#13785,.F.);
#18748=ORIENTED_EDGE('',*,*,#13789,.F.);
#18749=ORIENTED_EDGE('',*,*,#13790,.T.);
#18750=ORIENTED_EDGE('',*,*,#13752,.F.);
#18751=ORIENTED_EDGE('',*,*,#13788,.F.);
#18752=ORIENTED_EDGE('',*,*,#13791,.F.);
#18753=ORIENTED_EDGE('',*,*,#13786,.T.);
#18754=ORIENTED_EDGE('',*,*,#13753,.F.);
#18755=ORIENTED_EDGE('',*,*,#13790,.F.);
#18756=ORIENTED_EDGE('',*,*,#13791,.T.);
#18757=ORIENTED_EDGE('',*,*,#13789,.T.);
#18758=ORIENTED_EDGE('',*,*,#13787,.T.);
#18759=ORIENTED_EDGE('',*,*,#13784,.T.);
#18760=ORIENTED_EDGE('',*,*,#13758,.F.);
#18761=ORIENTED_EDGE('',*,*,#13792,.T.);
#18762=ORIENTED_EDGE('',*,*,#13793,.T.);
#18763=ORIENTED_EDGE('',*,*,#13794,.F.);
#18764=ORIENTED_EDGE('',*,*,#13761,.F.);
#18765=ORIENTED_EDGE('',*,*,#13795,.T.);
#18766=ORIENTED_EDGE('',*,*,#13796,.T.);
#18767=ORIENTED_EDGE('',*,*,#13792,.F.);
#18768=ORIENTED_EDGE('',*,*,#13760,.F.);
#18769=ORIENTED_EDGE('',*,*,#13797,.T.);
#18770=ORIENTED_EDGE('',*,*,#13798,.T.);
#18771=ORIENTED_EDGE('',*,*,#13795,.F.);
#18772=ORIENTED_EDGE('',*,*,#13759,.F.);
#18773=ORIENTED_EDGE('',*,*,#13794,.T.);
#18774=ORIENTED_EDGE('',*,*,#13799,.T.);
#18775=ORIENTED_EDGE('',*,*,#13797,.F.);
#18776=ORIENTED_EDGE('',*,*,#13799,.F.);
#18777=ORIENTED_EDGE('',*,*,#13793,.F.);
#18778=ORIENTED_EDGE('',*,*,#13796,.F.);
#18779=ORIENTED_EDGE('',*,*,#13798,.F.);
#18780=ORIENTED_EDGE('',*,*,#13731,.F.);
#18781=ORIENTED_EDGE('',*,*,#13721,.T.);
#18782=ORIENTED_EDGE('',*,*,#13763,.F.);
#18783=ORIENTED_EDGE('',*,*,#13743,.T.);
#23753=ADVANCED_FACE('',(#3000),#1458,.T.);
#23754=ADVANCED_FACE('',(#3001),#1459,.T.);
#23755=ADVANCED_FACE('',(#3002),#1460,.T.);
#23756=ADVANCED_FACE('',(#3003),#1461,.T.);
#23757=ADVANCED_FACE('',(#3004),#1462,.T.);
#23758=ADVANCED_FACE('',(#3005),#1463,.T.);
#23759=ADVANCED_FACE('',(#3006),#1464,.T.);
#23760=ADVANCED_FACE('',(#3007,#1232),#1465,.T.);
#23761=ADVANCED_FACE('',(#3008),#1466,.T.);
#23762=ADVANCED_FACE('',(#3009),#1467,.F.);
#23763=ADVANCED_FACE('',(#3010),#1468,.T.);
#23764=ADVANCED_FACE('',(#3011,#1233),#1469,.F.);
#23765=ADVANCED_FACE('',(#3012),#1470,.T.);
#23766=ADVANCED_FACE('',(#3013),#1471,.T.);
#23767=ADVANCED_FACE('',(#3014,#1234,#1235,#1236),#1472,.T.);
#23768=ADVANCED_FACE('',(#3015),#1473,.T.);
#23769=ADVANCED_FACE('',(#3016),#1474,.F.);
#23770=ADVANCED_FACE('',(#3017),#2178,.F.);
#23771=ADVANCED_FACE('',(#3018),#2179,.F.);
#23772=ADVANCED_FACE('',(#3019),#1475,.T.);
#23773=ADVANCED_FACE('',(#3020,#1237,#1238),#1476,.T.);
#23774=ADVANCED_FACE('',(#3021),#1477,.T.);
#23775=ADVANCED_FACE('',(#3022),#1478,.T.);
#23776=ADVANCED_FACE('',(#3023),#1479,.F.);
#23777=ADVANCED_FACE('',(#3024),#1480,.F.);
#23778=ADVANCED_FACE('',(#3025),#1481,.F.);
#23779=ADVANCED_FACE('',(#3026),#1482,.F.);
#23780=ADVANCED_FACE('',(#3027),#1483,.F.);
#23781=ADVANCED_FACE('',(#3028),#1484,.T.);
#23782=ADVANCED_FACE('',(#3029),#1485,.F.);
#23783=ADVANCED_FACE('',(#3030),#1486,.F.);
#23784=ADVANCED_FACE('',(#3031),#1487,.F.);
#23785=ADVANCED_FACE('',(#3032),#1488,.F.);
#23786=ADVANCED_FACE('',(#3033),#1489,.F.);
#23787=ADVANCED_FACE('',(#3034),#1490,.T.);
#24539=CLOSED_SHELL('',(#23753,#23754,#23755,#23756,#23757,#23758,#23759,
#23760,#23761,#23762,#23763,#23764,#23765,#23766,#23767,#23768,#23769,#23770,
#23771,#23772,#23773,#23774,#23775,#23776,#23777,#23778,#23779,#23780,#23781,
#23782,#23783,#23784,#23785,#23786,#23787));
#26022=AXIS2_PLACEMENT_3D('',#37260,#30382,#30383);
#26023=AXIS2_PLACEMENT_3D('',#37261,#30384,#30385);
#26024=AXIS2_PLACEMENT_3D('',#37270,#30390,#30391);
#26025=AXIS2_PLACEMENT_3D('',#37276,#30395,#30396);
#26026=AXIS2_PLACEMENT_3D('',#37304,#30411,#30412);
#26027=AXIS2_PLACEMENT_3D('',#37310,#30416,#30417);
#26028=AXIS2_PLACEMENT_3D('',#37314,#30420,#30421);
#26029=AXIS2_PLACEMENT_3D('',#37337,#30434,#30435);
#26030=AXIS2_PLACEMENT_3D('',#37339,#30437,#30438);
#26031=AXIS2_PLACEMENT_3D('',#37349,#30444,#30445);
#26032=AXIS2_PLACEMENT_3D('',#37351,#30447,#30448);
#26033=AXIS2_PLACEMENT_3D('',#37353,#30450,#30451);
#26034=AXIS2_PLACEMENT_3D('',#37355,#30453,#30454);
#26035=AXIS2_PLACEMENT_3D('',#37365,#30460,#30461);
#26036=AXIS2_PLACEMENT_3D('',#37366,#30462,#30463);
#26037=AXIS2_PLACEMENT_3D('',#37369,#30466,#30467);
#26038=AXIS2_PLACEMENT_3D('',#37379,#30472,#30473);
#26039=AXIS2_PLACEMENT_3D('',#37381,#30474,#30475);
#26040=AXIS2_PLACEMENT_3D('',#37383,#30477,#30478);
#26041=AXIS2_PLACEMENT_3D('',#37385,#30480,#30481);
#26042=AXIS2_PLACEMENT_3D('',#37386,#30482,#30483);
#26043=AXIS2_PLACEMENT_3D('',#37388,#30484,#30485);
#26044=AXIS2_PLACEMENT_3D('',#37390,#30487,#30488);
#26045=AXIS2_PLACEMENT_3D('',#37392,#30489,#30490);
#26046=AXIS2_PLACEMENT_3D('',#37394,#30492,#30493);
#26047=AXIS2_PLACEMENT_3D('',#37400,#30497,#30498);
#26048=AXIS2_PLACEMENT_3D('',#37406,#30502,#30503);
#26049=AXIS2_PLACEMENT_3D('',#37409,#30506,#30507);
#26050=AXIS2_PLACEMENT_3D('',#37410,#30508,#30509);
#26051=AXIS2_PLACEMENT_3D('',#37411,#30510,#30511);
#26052=AXIS2_PLACEMENT_3D('',#37417,#30515,#30516);
#26053=AXIS2_PLACEMENT_3D('',#37421,#30519,#30520);
#26054=AXIS2_PLACEMENT_3D('',#37425,#30523,#30524);
#26055=AXIS2_PLACEMENT_3D('',#37427,#30526,#30527);
#26056=AXIS2_PLACEMENT_3D('',#37428,#30528,#30529);
#26057=AXIS2_PLACEMENT_3D('',#37434,#30533,#30534);
#26058=AXIS2_PLACEMENT_3D('',#37438,#30537,#30538);
#26059=AXIS2_PLACEMENT_3D('',#37442,#30541,#30542);
#26060=AXIS2_PLACEMENT_3D('',#37444,#30544,#30545);
#26061=AXIS2_PLACEMENT_3D('',#37445,#30546,#30547);
#30382=DIRECTION('axis',(0.,0.,1.));
#30383=DIRECTION('refdir',(1.,0.,0.));
#30384=DIRECTION('center_axis',(-0.707106781186544,0.,-0.707106781186551));
#30385=DIRECTION('ref_axis',(-0.707106781186551,0.,0.707106781186544));
#30386=DIRECTION('',(-0.707106781186551,0.,0.707106781186544));
#30387=DIRECTION('',(0.,1.,0.));
#30388=DIRECTION('',(0.707106781186551,0.,-0.707106781186544));
#30389=DIRECTION('',(0.,-1.,0.));
#30390=DIRECTION('center_axis',(-1.,0.,0.));
#30391=DIRECTION('ref_axis',(0.,-1.,0.));
#30392=DIRECTION('',(0.,0.,1.));
#30393=DIRECTION('',(0.,-1.,0.));
#30394=DIRECTION('',(0.,0.,1.));
#30395=DIRECTION('center_axis',(0.,-1.,0.));
#30396=DIRECTION('ref_axis',(1.,0.,0.));
#30397=DIRECTION('',(1.,0.,0.));
#30398=DIRECTION('',(-0.707106781186548,0.,0.707106781186548));
#30399=DIRECTION('',(0.,0.,1.));
#30400=DIRECTION('',(0.707106781186548,0.,0.707106781186547));
#30401=DIRECTION('',(1.,0.,0.));
#30402=DIRECTION('',(0.707106781186548,0.,0.707106781186548));
#30403=DIRECTION('',(0.,0.,1.));
#30404=DIRECTION('',(-0.707106781186547,0.,0.707106781186548));
#30405=DIRECTION('',(1.,0.,0.));
#30406=DIRECTION('',(-0.707106781186548,0.,0.707106781186547));
#30407=DIRECTION('',(0.,0.,-1.));
#30408=DIRECTION('',(0.707106781186548,0.,0.707106781186547));
#30409=DIRECTION('',(-1.,0.,0.));
#30410=DIRECTION('',(0.707106781186548,0.,0.707106781186547));
#30411=DIRECTION('center_axis',(-0.707106781186548,0.,0.707106781186548));
#30412=DIRECTION('ref_axis',(0.707106781186548,0.,0.707106781186548));
#30413=DIRECTION('',(0.,1.,0.));
#30414=DIRECTION('',(-0.707106781186548,0.,-0.707106781186548));
#30415=DIRECTION('',(0.,-1.,0.));
#30416=DIRECTION('center_axis',(-1.,0.,0.));
#30417=DIRECTION('ref_axis',(0.,-1.,0.));
#30418=DIRECTION('',(0.,0.,1.));
#30419=DIRECTION('',(0.,1.,0.));
#30420=DIRECTION('center_axis',(0.,1.,0.));
#30421=DIRECTION('ref_axis',(-1.,0.,0.));
#30422=DIRECTION('',(-0.707106781186548,0.,-0.707106781186547));
#30423=DIRECTION('',(1.,0.,0.));
#30424=DIRECTION('',(-0.707106781186548,0.,-0.707106781186547));
#30425=DIRECTION('',(0.,0.,1.));
#30426=DIRECTION('',(0.707106781186548,0.,-0.707106781186547));
#30427=DIRECTION('',(-1.,0.,0.));
#30428=DIRECTION('',(0.707106781186547,0.,-0.707106781186548));
#30429=DIRECTION('',(-1.,0.,0.));
#30430=DIRECTION('',(-0.707106781186548,0.,-0.707106781186547));
#30431=DIRECTION('',(0.,0.,1.));
#30432=DIRECTION('',(0.707106781186548,0.,-0.707106781186548));
#30433=DIRECTION('',(-1.,0.,0.));
#30434=DIRECTION('center_axis',(-0.707106781186547,0.,0.707106781186548));
#30435=DIRECTION('ref_axis',(0.707106781186548,0.,0.707106781186547));
#30436=DIRECTION('',(0.,1.,0.));
#30437=DIRECTION('center_axis',(0.,0.,1.));
#30438=DIRECTION('ref_axis',(1.,0.,0.));
#30439=DIRECTION('',(0.,-1.,0.));
#30440=DIRECTION('',(1.,0.,0.));
#30441=DIRECTION('',(0.,-1.,0.));
#30442=DIRECTION('',(-1.,0.,0.));
#30443=DIRECTION('',(0.,1.,0.));
#30444=DIRECTION('center_axis',(-0.707106781186547,0.,0.707106781186548));
#30445=DIRECTION('ref_axis',(0.707106781186548,0.,0.707106781186547));
#30446=DIRECTION('',(0.,1.,0.));
#30447=DIRECTION('center_axis',(1.,0.,0.));
#30448=DIRECTION('ref_axis',(0.,1.,0.));
#30449=DIRECTION('',(0.,-1.,0.));
#30450=DIRECTION('center_axis',(-0.707106781186548,0.,-0.707106781186547));
#30451=DIRECTION('ref_axis',(-0.707106781186547,0.,0.707106781186548));
#30452=DIRECTION('',(0.,-1.,0.));
#30453=DIRECTION('center_axis',(0.,0.,1.));
#30454=DIRECTION('ref_axis',(1.,0.,0.));
#30455=DIRECTION('',(0.,1.,0.));
#30456=DIRECTION('',(-1.,0.,0.));
#30457=DIRECTION('',(0.,-1.,0.));
#30458=DIRECTION('',(1.,0.,0.));
#30459=DIRECTION('',(0.,1.,0.));
#30460=DIRECTION('center_axis',(-0.707106781186547,0.,-0.707106781186548));
#30461=DIRECTION('ref_axis',(-0.707106781186548,0.,0.707106781186547));
#30462=DIRECTION('center_axis',(-0.707106781186547,0.,0.707106781186548));
#30463=DIRECTION('ref_axis',(0.707106781186548,0.,0.707106781186547));
#30464=DIRECTION('',(0.,1.,0.));
#30465=DIRECTION('',(0.,-1.,0.));
#30466=DIRECTION('center_axis',(-1.,0.,0.));
#30467=DIRECTION('ref_axis',(0.,-1.,0.));
#30468=DIRECTION('',(0.,-1.,0.));
#30469=DIRECTION('',(0.,0.,1.));
#30470=DIRECTION('',(0.,-1.,0.));
#30471=DIRECTION('',(0.,0.,1.));
#30472=DIRECTION('center_axis',(1.,0.,0.));
#30473=DIRECTION('ref_axis',(0.,-1.,0.));
#30474=DIRECTION('center_axis',(1.,0.,0.));
#30475=DIRECTION('ref_axis',(0.,-1.,0.));
#30476=DIRECTION('',(0.,-1.,0.));
#30477=DIRECTION('center_axis',(-0.707106781186548,0.,-0.707106781186548));
#30478=DIRECTION('ref_axis',(-0.707106781186548,0.,0.707106781186548));
#30479=DIRECTION('',(0.,1.,0.));
#30480=DIRECTION('center_axis',(0.,0.,1.));
#30481=DIRECTION('ref_axis',(1.,0.,0.));
#30482=DIRECTION('center_axis',(-1.,0.,0.));
#30483=DIRECTION('ref_axis',(0.,-1.,0.));
#30484=DIRECTION('center_axis',(-1.,0.,0.));
#30485=DIRECTION('ref_axis',(0.,-1.,0.));
#30486=DIRECTION('',(-1.,0.,0.));
#30487=DIRECTION('center_axis',(-1.,0.,0.));
#30488=DIRECTION('ref_axis',(0.,-1.,0.));
#30489=DIRECTION('center_axis',(-1.,0.,0.));
#30490=DIRECTION('ref_axis',(0.,-1.,0.));
#30491=DIRECTION('',(-1.,0.,0.));
#30492=DIRECTION('center_axis',(0.,1.,0.));
#30493=DIRECTION('ref_axis',(-1.,0.,0.));
#30494=DIRECTION('',(-1.,0.,0.));
#30495=DIRECTION('',(-1.,0.,0.));
#30496=DIRECTION('',(0.,0.,1.));
#30497=DIRECTION('center_axis',(1.,0.,0.));
#30498=DIRECTION('ref_axis',(0.,1.,0.));
#30499=DIRECTION('',(0.,1.,0.));
#30500=DIRECTION('',(0.,1.,0.));
#30501=DIRECTION('',(0.,0.,1.));
#30502=DIRECTION('center_axis',(0.,-1.,0.));
#30503=DIRECTION('ref_axis',(1.,0.,0.));
#30504=DIRECTION('',(1.,0.,0.));
#30505=DIRECTION('',(1.,0.,0.));
#30506=DIRECTION('center_axis',(0.,0.,1.));
#30507=DIRECTION('ref_axis',(1.,0.,0.));
#30508=DIRECTION('center_axis',(0.,0.,1.));
#30509=DIRECTION('ref_axis',(1.,0.,0.));
#30510=DIRECTION('center_axis',(0.,1.,0.));
#30511=DIRECTION('ref_axis',(-1.,0.,0.));
#30512=DIRECTION('',(-1.,0.,0.));
#30513=DIRECTION('',(0.,0.,1.));
#30514=DIRECTION('',(0.,0.,1.));
#30515=DIRECTION('center_axis',(1.,0.,0.));
#30516=DIRECTION('ref_axis',(0.,1.,0.));
#30517=DIRECTION('',(0.,1.,0.));
#30518=DIRECTION('',(0.,0.,1.));
#30519=DIRECTION('center_axis',(0.,-1.,0.));
#30520=DIRECTION('ref_axis',(1.,0.,0.));
#30521=DIRECTION('',(1.,0.,0.));
#30522=DIRECTION('',(0.,0.,1.));
#30523=DIRECTION('center_axis',(-1.,0.,0.));
#30524=DIRECTION('ref_axis',(0.,-1.,0.));
#30525=DIRECTION('',(0.,-1.,0.));
#30526=DIRECTION('center_axis',(0.,0.,1.));
#30527=DIRECTION('ref_axis',(1.,0.,0.));
#30528=DIRECTION('center_axis',(0.,1.,0.));
#30529=DIRECTION('ref_axis',(-1.,0.,0.));
#30530=DIRECTION('',(0.,0.,1.));
#30531=DIRECTION('',(-1.,0.,0.));
#30532=DIRECTION('',(0.,0.,1.));
#30533=DIRECTION('center_axis',(1.,0.,0.));
#30534=DIRECTION('ref_axis',(0.,1.,0.));
#30535=DIRECTION('',(0.,0.,1.));
#30536=DIRECTION('',(0.,1.,0.));
#30537=DIRECTION('center_axis',(0.,-1.,0.));
#30538=DIRECTION('ref_axis',(1.,0.,0.));
#30539=DIRECTION('',(0.,0.,1.));
#30540=DIRECTION('',(1.,0.,0.));
#30541=DIRECTION('center_axis',(-1.,0.,0.));
#30542=DIRECTION('ref_axis',(0.,-1.,0.));
#30543=DIRECTION('',(0.,-1.,0.));
#30544=DIRECTION('center_axis',(0.,0.,1.));
#30545=DIRECTION('ref_axis',(1.,0.,0.));
#30546=DIRECTION('center_axis',(0.,0.,1.));
#30547=DIRECTION('ref_axis',(1.,0.,0.));
#37260=CARTESIAN_POINT('',(0.,0.,0.));
#37261=CARTESIAN_POINT('Origin',(1.46,0.15,-0.305));
#37262=CARTESIAN_POINT('',(1.47,-0.3,-0.315));
#37263=CARTESIAN_POINT('',(1.45,-0.3,-0.295));
#37264=CARTESIAN_POINT('',(1.46,-0.3,-0.305));
#37265=CARTESIAN_POINT('',(1.45,0.3,-0.295));
#37266=CARTESIAN_POINT('',(1.45,0.15,-0.295));
#37267=CARTESIAN_POINT('',(1.47,0.3,-0.315));
#37268=CARTESIAN_POINT('',(1.785,0.3,-0.63));
#37269=CARTESIAN_POINT('',(1.47,0.15,-0.315));
#37270=CARTESIAN_POINT('Origin',(1.45,0.3,-0.315));
#37271=CARTESIAN_POINT('',(1.45,-0.3,-0.17));
#37272=CARTESIAN_POINT('',(1.45,-0.3,-0.315));
#37273=CARTESIAN_POINT('',(1.45,0.3,-0.17));
#37274=CARTESIAN_POINT('',(1.45,0.15,-0.17));
#37275=CARTESIAN_POINT('',(1.45,0.3,-0.315));
#37276=CARTESIAN_POINT('Origin',(1.45,-0.3,-0.315));
#37277=CARTESIAN_POINT('',(2.73,-0.3,-0.315));
#37278=CARTESIAN_POINT('',(1.45,-0.3,-0.315));
#37279=CARTESIAN_POINT('',(2.75,-0.3,-0.335));
#37280=CARTESIAN_POINT('',(2.415,-0.3,1.11022302462516E-16));
#37281=CARTESIAN_POINT('',(2.75,-0.3,0.335));
#37282=CARTESIAN_POINT('',(2.75,-0.3,-0.315));
#37283=CARTESIAN_POINT('',(2.73,-0.3,0.315));
#37284=CARTESIAN_POINT('',(2.2575,-0.3,-0.1575));
#37285=CARTESIAN_POINT('',(1.47,-0.3,0.315));
#37286=CARTESIAN_POINT('',(1.45,-0.3,0.315));
#37287=CARTESIAN_POINT('',(1.45,-0.3,0.295));
#37288=CARTESIAN_POINT('',(1.3025,-0.3,0.1475));
#37289=CARTESIAN_POINT('',(1.45,-0.3,0.17));
#37290=CARTESIAN_POINT('',(1.45,-0.3,-0.315));
#37291=CARTESIAN_POINT('',(1.47,-0.3,0.15));
#37292=CARTESIAN_POINT('',(1.57625,-0.3,0.0437499999999999));
#37293=CARTESIAN_POINT('',(2.43,-0.3,0.15));
#37294=CARTESIAN_POINT('',(1.6875,-0.3,0.15));
#37295=CARTESIAN_POINT('',(2.45,-0.3,0.13));
#37296=CARTESIAN_POINT('',(2.30625,-0.3,0.27375));
#37297=CARTESIAN_POINT('',(2.45,-0.3,-0.13));
#37298=CARTESIAN_POINT('',(2.45,-0.3,-0.2325));
#37299=CARTESIAN_POINT('',(2.43,-0.3,-0.15));
#37300=CARTESIAN_POINT('',(2.14875,-0.3,-0.43125));
#37301=CARTESIAN_POINT('',(1.47,-0.3,-0.15));
#37302=CARTESIAN_POINT('',(1.6875,-0.3,-0.15));
#37303=CARTESIAN_POINT('',(1.41875,-0.3,-0.20125));
#37304=CARTESIAN_POINT('Origin',(1.46,0.15,0.305));
#37305=CARTESIAN_POINT('',(1.47,0.3,0.315));
#37306=CARTESIAN_POINT('',(1.47,0.15,0.315));
#37307=CARTESIAN_POINT('',(1.45,0.3,0.295));
#37308=CARTESIAN_POINT('',(1.6275,0.3,0.4725));
#37309=CARTESIAN_POINT('',(1.45,0.15,0.295));
#37310=CARTESIAN_POINT('Origin',(1.45,0.3,-0.315));
#37311=CARTESIAN_POINT('',(1.45,0.3,0.17));
#37312=CARTESIAN_POINT('',(1.45,0.3,-0.315));
#37313=CARTESIAN_POINT('',(1.45,0.15,0.17));
#37314=CARTESIAN_POINT('Origin',(2.75,0.3,-0.315));
#37315=CARTESIAN_POINT('',(1.47,0.3,-0.15));
#37316=CARTESIAN_POINT('',(1.74375,0.3,0.12375));
#37317=CARTESIAN_POINT('',(2.43,0.3,-0.15));
#37318=CARTESIAN_POINT('',(2.3375,0.3,-0.15));
#37319=CARTESIAN_POINT('',(2.45,0.3,-0.13));
#37320=CARTESIAN_POINT('',(2.47375,0.3,-0.10625));
#37321=CARTESIAN_POINT('',(2.45,0.3,0.13));
#37322=CARTESIAN_POINT('',(2.45,0.3,-0.2325));
#37323=CARTESIAN_POINT('',(2.43,0.3,0.15));
#37324=CARTESIAN_POINT('',(2.63125,0.3,-0.0512499999999997));
#37325=CARTESIAN_POINT('',(1.47,0.3,0.15));
#37326=CARTESIAN_POINT('',(2.3375,0.3,0.15));
#37327=CARTESIAN_POINT('',(1.90125,0.3,-0.28125));
#37328=CARTESIAN_POINT('',(2.73,0.3,0.315));
#37329=CARTESIAN_POINT('',(2.75,0.3,0.315));
#37330=CARTESIAN_POINT('',(2.75,0.3,0.335));
#37331=CARTESIAN_POINT('',(2.5825,0.3,0.1675));
#37332=CARTESIAN_POINT('',(2.75,0.3,-0.335));
#37333=CARTESIAN_POINT('',(2.75,0.3,-0.315));
#37334=CARTESIAN_POINT('',(2.73,0.3,-0.315));
#37335=CARTESIAN_POINT('',(2.74,0.3,-0.325));
#37336=CARTESIAN_POINT('',(2.75,0.3,-0.315));
#37337=CARTESIAN_POINT('Origin',(1.46,0.15,-0.16));
#37338=CARTESIAN_POINT('',(1.47,0.15,-0.15));
#37339=CARTESIAN_POINT('Origin',(1.925,0.,-0.15));
#37340=CARTESIAN_POINT('',(2.43,-0.175,-0.15));
#37341=CARTESIAN_POINT('',(1.65,0.05,-0.15));
#37342=CARTESIAN_POINT('',(1.75,0.05,-0.15));
#37343=CARTESIAN_POINT('',(1.8375,0.05,-0.15));
#37344=CARTESIAN_POINT('',(1.75,-0.05,-0.15));
#37345=CARTESIAN_POINT('',(1.75,-0.025,-0.15));
#37346=CARTESIAN_POINT('',(1.65,-0.05,-0.15));
#37347=CARTESIAN_POINT('',(1.7875,-0.05,-0.15));
#37348=CARTESIAN_POINT('',(1.65,0.025,-0.15));
#37349=CARTESIAN_POINT('Origin',(2.44,-0.175,-0.14));
#37350=CARTESIAN_POINT('',(2.45,-0.175,-0.13));
#37351=CARTESIAN_POINT('Origin',(2.45,-0.35,-0.15));
#37352=CARTESIAN_POINT('',(2.45,-0.175,0.13));
#37353=CARTESIAN_POINT('Origin',(1.46,0.15,0.16));
#37354=CARTESIAN_POINT('',(1.47,0.15,0.15));
#37355=CARTESIAN_POINT('Origin',(1.925,0.,0.15));
#37356=CARTESIAN_POINT('',(2.43,-0.175,0.15));
#37357=CARTESIAN_POINT('',(1.75,0.05,0.15));
#37358=CARTESIAN_POINT('',(1.65,0.05,0.15));
#37359=CARTESIAN_POINT('',(1.8375,0.05,0.15));
#37360=CARTESIAN_POINT('',(1.65,-0.05,0.15));
#37361=CARTESIAN_POINT('',(1.65,0.025,0.15));
#37362=CARTESIAN_POINT('',(1.75,-0.05,0.15));
#37363=CARTESIAN_POINT('',(1.7875,-0.05,0.15));
#37364=CARTESIAN_POINT('',(1.75,-0.025,0.15));
#37365=CARTESIAN_POINT('Origin',(2.44,-0.175,0.14));
#37366=CARTESIAN_POINT('Origin',(2.74,0.35,0.325));
#37367=CARTESIAN_POINT('',(2.75,0.35,0.335));
#37368=CARTESIAN_POINT('',(2.73,0.35,0.315));
#37369=CARTESIAN_POINT('Origin',(2.75,0.7,-0.385));
#37370=CARTESIAN_POINT('',(2.75,0.7,-0.385));
#37371=CARTESIAN_POINT('',(2.75,-0.7,-0.385));
#37372=CARTESIAN_POINT('',(2.75,0.7,-0.385));
#37373=CARTESIAN_POINT('',(2.75,-0.7,0.365));
#37374=CARTESIAN_POINT('',(2.75,-0.7,-0.385));
#37375=CARTESIAN_POINT('',(2.75,0.7,0.365));
#37376=CARTESIAN_POINT('',(2.75,0.7,0.365));
#37377=CARTESIAN_POINT('',(2.75,0.7,-0.385));
#37378=CARTESIAN_POINT('',(2.75,0.61,1.10218211923262E-17));
#37379=CARTESIAN_POINT('Origin',(2.75,0.52,0.));
#37380=CARTESIAN_POINT('',(2.75,-0.43,1.10218211923262E-17));
#37381=CARTESIAN_POINT('Origin',(2.75,-0.52,0.));
#37382=CARTESIAN_POINT('',(2.75,0.35,-0.335));
#37383=CARTESIAN_POINT('Origin',(2.74,0.35,-0.325));
#37384=CARTESIAN_POINT('',(2.73,0.35,-0.315));
#37385=CARTESIAN_POINT('Origin',(2.1,0.,-0.315));
#37386=CARTESIAN_POINT('Origin',(2.805,-0.52,0.));
#37387=CARTESIAN_POINT('',(2.91,-0.43,-1.10218211923262E-17));
#37388=CARTESIAN_POINT('Origin',(2.91,-0.52,0.));
#37389=CARTESIAN_POINT('',(2.805,-0.43,-1.10218211923262E-17));
#37390=CARTESIAN_POINT('Origin',(2.805,0.52,0.));
#37391=CARTESIAN_POINT('',(2.91,0.61,-1.10218211923262E-17));
#37392=CARTESIAN_POINT('Origin',(2.91,0.52,0.));
#37393=CARTESIAN_POINT('',(2.805,0.61,-1.10218211923262E-17));
#37394=CARTESIAN_POINT('Origin',(2.91,0.7,-0.385));
#37395=CARTESIAN_POINT('',(2.91,0.7,-0.385));
#37396=CARTESIAN_POINT('',(2.91,0.7,-0.385));
#37397=CARTESIAN_POINT('',(2.91,0.7,0.365));
#37398=CARTESIAN_POINT('',(2.91,0.7,0.365));
#37399=CARTESIAN_POINT('',(2.91,0.7,-0.385));
#37400=CARTESIAN_POINT('Origin',(2.91,-0.7,-0.385));
#37401=CARTESIAN_POINT('',(2.91,-0.7,-0.385));
#37402=CARTESIAN_POINT('',(2.91,-0.7,-0.385));
#37403=CARTESIAN_POINT('',(2.91,-0.7,0.365));
#37404=CARTESIAN_POINT('',(2.91,-0.7,0.365));
#37405=CARTESIAN_POINT('',(2.91,-0.7,-0.385));
#37406=CARTESIAN_POINT('Origin',(2.75,-0.7,-0.385));
#37407=CARTESIAN_POINT('',(2.75,-0.7,-0.385));
#37408=CARTESIAN_POINT('',(2.75,-0.7,0.365));
#37409=CARTESIAN_POINT('Origin',(2.83,0.,0.365));
#37410=CARTESIAN_POINT('Origin',(2.83,0.,-0.385));
#37411=CARTESIAN_POINT('Origin',(1.75,0.05,-0.19));
#37412=CARTESIAN_POINT('',(1.75,0.05,-0.19));
#37413=CARTESIAN_POINT('',(1.65,0.05,-0.19));
#37414=CARTESIAN_POINT('',(1.75,0.05,-0.19));
#37415=CARTESIAN_POINT('',(1.75,0.05,-0.19));
#37416=CARTESIAN_POINT('',(1.65,0.05,-0.19));
#37417=CARTESIAN_POINT('Origin',(1.75,-0.05,-0.19));
#37418=CARTESIAN_POINT('',(1.75,-0.05,-0.19));
#37419=CARTESIAN_POINT('',(1.75,-0.05,-0.19));
#37420=CARTESIAN_POINT('',(1.75,-0.05,-0.19));
#37421=CARTESIAN_POINT('Origin',(1.65,-0.05,-0.19));
#37422=CARTESIAN_POINT('',(1.65,-0.05,-0.19));
#37423=CARTESIAN_POINT('',(1.65,-0.05,-0.19));
#37424=CARTESIAN_POINT('',(1.65,-0.05,-0.19));
#37425=CARTESIAN_POINT('Origin',(1.65,0.05,-0.19));
#37426=CARTESIAN_POINT('',(1.65,0.05,-0.19));
#37427=CARTESIAN_POINT('Origin',(1.7,0.,-0.19));
#37428=CARTESIAN_POINT('Origin',(1.75,0.05,0.15));
#37429=CARTESIAN_POINT('',(1.75,0.05,0.19));
#37430=CARTESIAN_POINT('',(1.75,0.05,0.15));
#37431=CARTESIAN_POINT('',(1.65,0.05,0.19));
#37432=CARTESIAN_POINT('',(1.75,0.05,0.19));
#37433=CARTESIAN_POINT('',(1.65,0.05,0.15));
#37434=CARTESIAN_POINT('Origin',(1.75,-0.05,0.15));
#37435=CARTESIAN_POINT('',(1.75,-0.05,0.19));
#37436=CARTESIAN_POINT('',(1.75,-0.05,0.15));
#37437=CARTESIAN_POINT('',(1.75,-0.05,0.19));
#37438=CARTESIAN_POINT('Origin',(1.65,-0.05,0.15));
#37439=CARTESIAN_POINT('',(1.65,-0.05,0.19));
#37440=CARTESIAN_POINT('',(1.65,-0.05,0.15));
#37441=CARTESIAN_POINT('',(1.65,-0.05,0.19));
#37442=CARTESIAN_POINT('Origin',(1.65,0.05,0.15));
#37443=CARTESIAN_POINT('',(1.65,0.05,0.19));
#37444=CARTESIAN_POINT('Origin',(1.7,0.,0.19));
#37445=CARTESIAN_POINT('Origin',(2.1,0.,0.315));
#54970=UNCERTAINTY_MEASURE_WITH_UNIT(LENGTH_MEASURE(0.001),#55003,
'DISTANCE_ACCURACY_VALUE',
'Maximum model space distance between geometric entities at asserted c
onnectivities');
#54980=UNCERTAINTY_MEASURE_WITH_UNIT(LENGTH_MEASURE(0.001),#55003,
'DISTANCE_ACCURACY_VALUE',
'Maximum model space distance between geometric entities at asserted c
onnectivities');
#54992=(
GEOMETRIC_REPRESENTATION_CONTEXT(3)
GLOBAL_UNCERTAINTY_ASSIGNED_CONTEXT((#54970))
GLOBAL_UNIT_ASSIGNED_CONTEXT((#55003,#55005,#55006))
REPRESENTATION_CONTEXT('','3D')
);
#55002=(
GEOMETRIC_REPRESENTATION_CONTEXT(3)
GLOBAL_UNCERTAINTY_ASSIGNED_CONTEXT((#54980))
GLOBAL_UNIT_ASSIGNED_CONTEXT((#55003,#55005,#55006))
REPRESENTATION_CONTEXT('','3D')
);
#55003=(
LENGTH_UNIT()
NAMED_UNIT(*)
SI_UNIT(.CENTI.,.METRE.)
);
#55005=(
NAMED_UNIT(*)
PLANE_ANGLE_UNIT()
SI_UNIT($,.RADIAN.)
);
#55006=(
NAMED_UNIT(*)
SI_UNIT($,.STERADIAN.)
SOLID_ANGLE_UNIT()
);
#55018=SHAPE_DEFINITION_REPRESENTATION(#55039,#55114);
#55039=PRODUCT_DEFINITION_SHAPE('',$,#55136);
#55114=SHAPE_REPRESENTATION('',(#26022),#54992);
#55124=PRODUCT_DEFINITION_CONTEXT('part definition',#55189,'design');
#55136=PRODUCT_DEFINITION('2026-10-18-23-36-29-833',
'11_Optoelectronic_Slot_Sensor_PCB',#55157,#55124);
#55157=PRODUCT_DEFINITION_FORMATION('',$,#55202);
#55189=APPLICATION_CONTEXT(
'Core Data for Automotive Mechanical Design Process');
#55190=PRODUCT_CONTEXT('part definition',#55189,'mechanical');
#55202=PRODUCT('2026-10-18-23-36-29-833',
'11_Optoelectronic_Slot_Sensor_PCB',$,(#55190));
#55373=COLOUR_RGB('Sky Blue',0.24,0.69,0.87);
#55374=FILL_AREA_STYLE_COLOUR('',#55373);
#55375=FILL_AREA_STYLE('',(#55374));
#55376=SURFACE_STYLE_FILL_AREA(#55375);
#55377=SURFACE_SIDE_STYLE('',(#55376));
#55378=SURFACE_STYLE_USAGE(.BOTH.,#55377);
#55379=PRESENTATION_STYLE_ASSIGNMENT((#55378));
ENDSEC;
END-ISO-10303-21;
